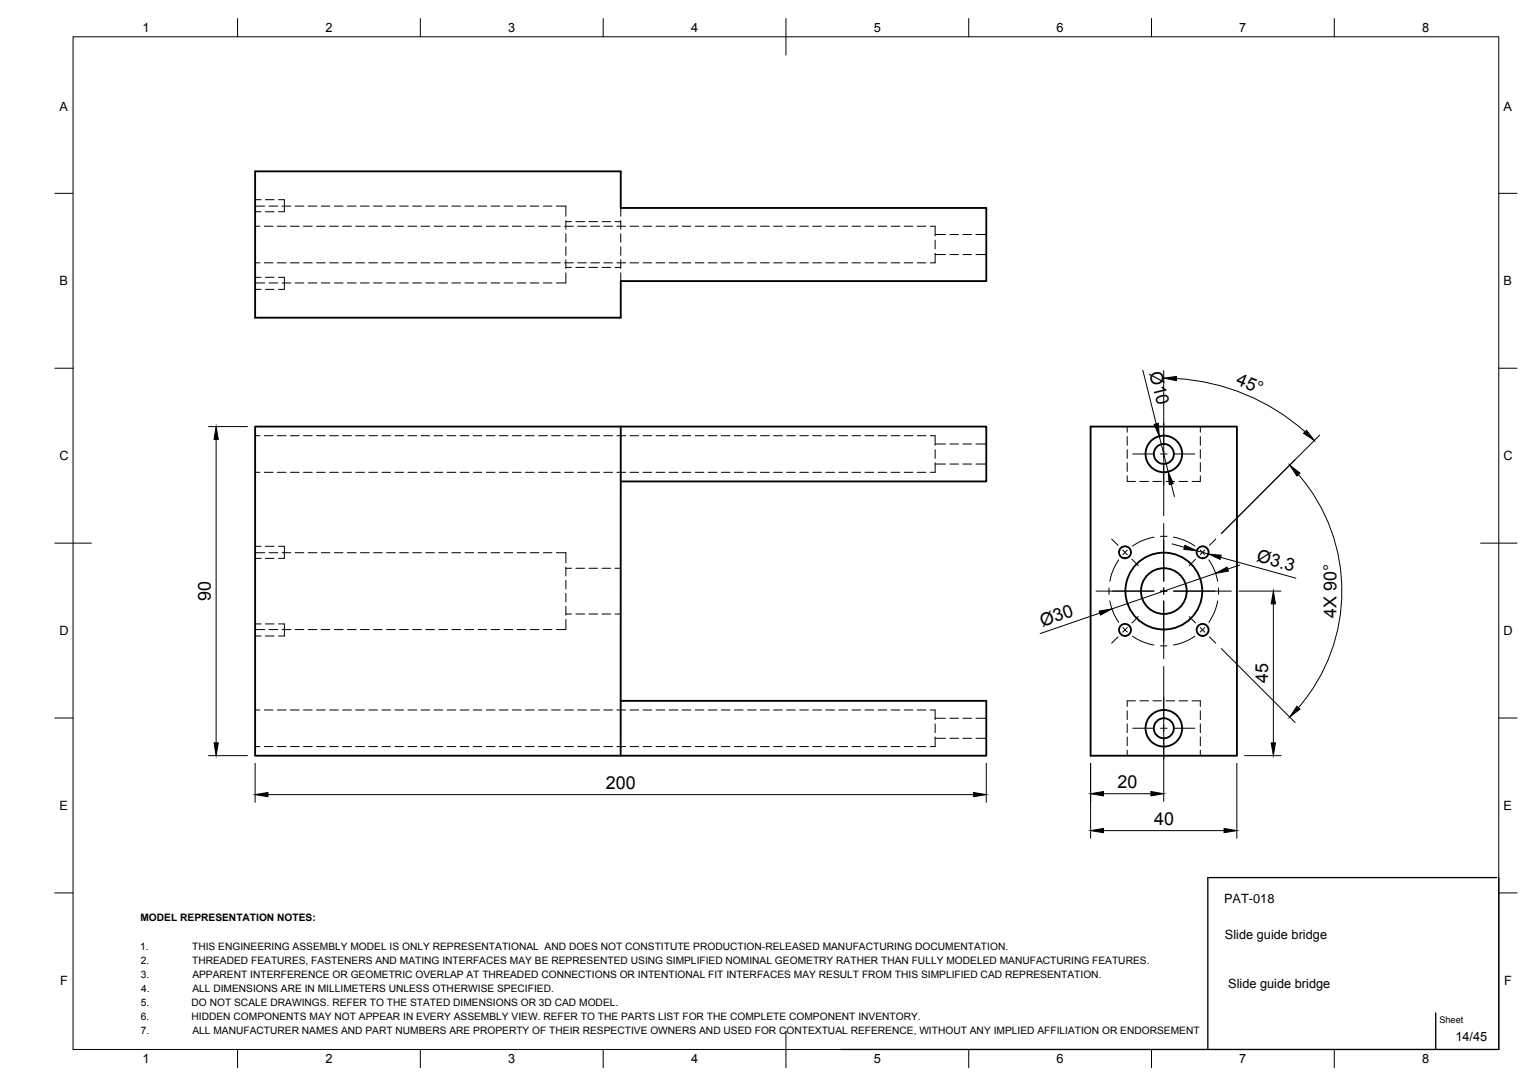
ISO-10303-21;
HEADER;
/* Generated by software containing ST-Developer
 * from STEP Tools, Inc. (www.steptools.com) 
 */

FILE_DESCRIPTION(
/* description */ ('Cam-driven reciprocating slide'),
/* implementation_level */ '2;1');

FILE_NAME(
/* name */ 'Slide guide bridge.step',
/* time_stamp */ '2026-10-28T03:25:20-07:00',
/* author */ (''),
/* organization */ (''),
/* preprocessor_version */ 'ST-DEVELOPER v20.2',
/* originating_system */ 'Autodesk Translation Framework v15.17.0.0',
/* authorisation */ '');

FILE_SCHEMA (('AUTOMOTIVE_DESIGN { 1 0 10303 214 3 1 1 }'));
ENDSEC;

DATA;
#10=MECHANICAL_DESIGN_GEOMETRIC_PRESENTATION_REPRESENTATION('',(#431),#13277);
#357=SHAPE_REPRESENTATION_RELATIONSHIP('SRR','None',#13450,#394);
#394=ADVANCED_BREP_SHAPE_REPRESENTATION('',(#475),#13245);
#431=STYLED_ITEM('',(#13713),#475);
#475=MANIFOLD_SOLID_BREP('Body1',#6407);
#592=FACE_BOUND('',#1478,.T.);
#593=FACE_BOUND('',#1482,.T.);
#594=FACE_BOUND('',#1486,.T.);
#595=FACE_BOUND('',#1489,.T.);
#596=FACE_BOUND('',#1495,.T.);
#597=FACE_BOUND('',#1503,.T.);
#598=FACE_BOUND('',#1504,.T.);
#599=FACE_BOUND('',#1505,.T.);
#600=FACE_BOUND('',#1506,.T.);
#601=FACE_BOUND('',#1507,.T.);
#602=FACE_BOUND('',#1508,.T.);
#603=FACE_BOUND('',#1509,.T.);
#604=FACE_BOUND('',#1511,.T.);
#736=PLANE('',#7067);
#737=PLANE('',#7071);
#738=PLANE('',#7075);
#739=PLANE('',#7079);
#740=PLANE('',#7083);
#741=PLANE('',#7090);
#742=PLANE('',#7097);
#743=PLANE('',#7101);
#744=PLANE('',#7102);
#745=PLANE('',#7103);
#746=PLANE('',#7104);
#747=PLANE('',#7105);
#748=PLANE('',#7106);
#749=PLANE('',#7107);
#750=PLANE('',#7108);
#751=PLANE('',#7109);
#752=PLANE('',#7110);
#753=PLANE('',#7111);
#754=PLANE('',#7112);
#755=PLANE('',#7113);
#756=PLANE('',#7114);
#1004=FACE_OUTER_BOUND('',#1468,.T.);
#1005=FACE_OUTER_BOUND('',#1469,.T.);
#1006=FACE_OUTER_BOUND('',#1470,.T.);
#1007=FACE_OUTER_BOUND('',#1471,.T.);
#1008=FACE_OUTER_BOUND('',#1472,.T.);
#1009=FACE_OUTER_BOUND('',#1473,.T.);
#1010=FACE_OUTER_BOUND('',#1474,.T.);
#1011=FACE_OUTER_BOUND('',#1475,.T.);
#1012=FACE_OUTER_BOUND('',#1476,.T.);
#1013=FACE_OUTER_BOUND('',#1477,.T.);
#1014=FACE_OUTER_BOUND('',#1479,.T.);
#1015=FACE_OUTER_BOUND('',#1480,.T.);
#1016=FACE_OUTER_BOUND('',#1481,.T.);
#1017=FACE_OUTER_BOUND('',#1483,.T.);
#1018=FACE_OUTER_BOUND('',#1484,.T.);
#1019=FACE_OUTER_BOUND('',#1485,.T.);
#1020=FACE_OUTER_BOUND('',#1487,.T.);
#1021=FACE_OUTER_BOUND('',#1488,.T.);
#1022=FACE_OUTER_BOUND('',#1490,.T.);
#1023=FACE_OUTER_BOUND('',#1491,.T.);
#1024=FACE_OUTER_BOUND('',#1492,.T.);
#1025=FACE_OUTER_BOUND('',#1493,.T.);
#1026=FACE_OUTER_BOUND('',#1494,.T.);
#1027=FACE_OUTER_BOUND('',#1496,.T.);
#1028=FACE_OUTER_BOUND('',#1497,.T.);
#1029=FACE_OUTER_BOUND('',#1498,.T.);
#1030=FACE_OUTER_BOUND('',#1499,.T.);
#1031=FACE_OUTER_BOUND('',#1500,.T.);
#1032=FACE_OUTER_BOUND('',#1501,.T.);
#1033=FACE_OUTER_BOUND('',#1502,.T.);
#1034=FACE_OUTER_BOUND('',#1510,.T.);
#1468=EDGE_LOOP('',(#4816,#4817,#4818,#4819));
#1469=EDGE_LOOP('',(#4820));
#1470=EDGE_LOOP('',(#4821,#4822,#4823,#4824));
#1471=EDGE_LOOP('',(#4825));
#1472=EDGE_LOOP('',(#4826,#4827,#4828,#4829));
#1473=EDGE_LOOP('',(#4830));
#1474=EDGE_LOOP('',(#4831,#4832,#4833,#4834));
#1475=EDGE_LOOP('',(#4835));
#1476=EDGE_LOOP('',(#4836,#4837,#4838,#4839));
#1477=EDGE_LOOP('',(#4840));
#1478=EDGE_LOOP('',(#4841));
#1479=EDGE_LOOP('',(#4842,#4843,#4844,#4845));
#1480=EDGE_LOOP('',(#4846,#4847,#4848,#4849));
#1481=EDGE_LOOP('',(#4850));
#1482=EDGE_LOOP('',(#4851));
#1483=EDGE_LOOP('',(#4852,#4853,#4854,#4855));
#1484=EDGE_LOOP('',(#4856,#4857,#4858,#4859));
#1485=EDGE_LOOP('',(#4860));
#1486=EDGE_LOOP('',(#4861));
#1487=EDGE_LOOP('',(#4862,#4863,#4864,#4865));
#1488=EDGE_LOOP('',(#4866,#4867,#4868,#4869,#4870,#4871,#4872,#4873,#4874,
#4875,#4876,#4877));
#1489=EDGE_LOOP('',(#4878));
#1490=EDGE_LOOP('',(#4879,#4880,#4881,#4882));
#1491=EDGE_LOOP('',(#4883,#4884,#4885,#4886));
#1492=EDGE_LOOP('',(#4887,#4888,#4889,#4890));
#1493=EDGE_LOOP('',(#4891,#4892,#4893,#4894));
#1494=EDGE_LOOP('',(#4895,#4896,#4897,#4898));
#1495=EDGE_LOOP('',(#4899));
#1496=EDGE_LOOP('',(#4900,#4901,#4902,#4903,#4904,#4905,#4906,#4907));
#1497=EDGE_LOOP('',(#4908,#4909,#4910,#4911));
#1498=EDGE_LOOP('',(#4912,#4913,#4914,#4915));
#1499=EDGE_LOOP('',(#4916,#4917,#4918,#4919));
#1500=EDGE_LOOP('',(#4920,#4921,#4922,#4923));
#1501=EDGE_LOOP('',(#4924,#4925,#4926,#4927,#4928,#4929,#4930,#4931));
#1502=EDGE_LOOP('',(#4932,#4933,#4934,#4935));
#1503=EDGE_LOOP('',(#4936));
#1504=EDGE_LOOP('',(#4937));
#1505=EDGE_LOOP('',(#4938));
#1506=EDGE_LOOP('',(#4939));
#1507=EDGE_LOOP('',(#4940));
#1508=EDGE_LOOP('',(#4941));
#1509=EDGE_LOOP('',(#4942));
#1510=EDGE_LOOP('',(#4943,#4944,#4945,#4946));
#1511=EDGE_LOOP('',(#4947));
#1977=LINE('',#10259,#2416);
#1978=LINE('',#10266,#2417);
#1979=LINE('',#10273,#2418);
#1980=LINE('',#10280,#2419);
#1981=LINE('',#10287,#2420);
#1982=LINE('',#10295,#2421);
#1983=LINE('',#10300,#2422);
#1984=LINE('',#10308,#2423);
#1985=LINE('',#10313,#2424);
#1986=LINE('',#10321,#2425);
#1987=LINE('',#10325,#2426);
#1988=LINE('',#10327,#2427);
#1989=LINE('',#10329,#2428);
#1990=LINE('',#10331,#2429);
#1991=LINE('',#10333,#2430);
#1992=LINE('',#10335,#2431);
#1993=LINE('',#10337,#2432);
#1994=LINE('',#10339,#2433);
#1995=LINE('',#10341,#2434);
#1996=LINE('',#10343,#2435);
#1997=LINE('',#10345,#2436);
#1998=LINE('',#10346,#2437);
#1999=LINE('',#10350,#2438);
#2000=LINE('',#10351,#2439);
#2001=LINE('',#10352,#2440);
#2002=LINE('',#10356,#2441);
#2003=LINE('',#10357,#2442);
#2004=LINE('',#10358,#2443);
#2005=LINE('',#10361,#2444);
#2006=LINE('',#10363,#2445);
#2007=LINE('',#10364,#2446);
#2008=LINE('',#10367,#2447);
#2009=LINE('',#10368,#2448);
#2010=LINE('',#10371,#2449);
#2011=LINE('',#10372,#2450);
#2012=LINE('',#10374,#2451);
#2013=LINE('',#10375,#2452);
#2014=LINE('',#10379,#2453);
#2015=LINE('',#10381,#2454);
#2016=LINE('',#10382,#2455);
#2017=LINE('',#10385,#2456);
#2018=LINE('',#10386,#2457);
#2019=LINE('',#10389,#2458);
#2020=LINE('',#10390,#2459);
#2021=LINE('',#10392,#2460);
#2022=LINE('',#10393,#2461);
#2416=VECTOR('',#8239,0.165);
#2417=VECTOR('',#8248,0.165);
#2418=VECTOR('',#8257,0.165);
#2419=VECTOR('',#8266,0.165);
#2420=VECTOR('',#8275,1.05);
#2421=VECTOR('',#8286,0.625);
#2422=VECTOR('',#8291,0.5);
#2423=VECTOR('',#8302,0.275);
#2424=VECTOR('',#8307,0.5);
#2425=VECTOR('',#8318,0.275);
#2426=VECTOR('',#8321,1.);
#2427=VECTOR('',#8322,1.);
#2428=VECTOR('',#8323,1.);
#2429=VECTOR('',#8324,1.);
#2430=VECTOR('',#8325,1.);
#2431=VECTOR('',#8326,1.);
#2432=VECTOR('',#8327,1.);
#2433=VECTOR('',#8328,1.);
#2434=VECTOR('',#8329,1.);
#2435=VECTOR('',#8330,1.);
#2436=VECTOR('',#8331,1.);
#2437=VECTOR('',#8332,1.);
#2438=VECTOR('',#8335,1.);
#2439=VECTOR('',#8336,1.);
#2440=VECTOR('',#8337,1.);
#2441=VECTOR('',#8340,1.);
#2442=VECTOR('',#8341,1.);
#2443=VECTOR('',#8342,1.);
#2444=VECTOR('',#8345,1.);
#2445=VECTOR('',#8346,1.);
#2446=VECTOR('',#8347,1.);
#2447=VECTOR('',#8350,1.);
#2448=VECTOR('',#8351,1.);
#2449=VECTOR('',#8354,1.);
#2450=VECTOR('',#8355,1.);
#2451=VECTOR('',#8358,1.);
#2452=VECTOR('',#8359,1.);
#2453=VECTOR('',#8364,1.);
#2454=VECTOR('',#8365,1.);
#2455=VECTOR('',#8366,1.);
#2456=VECTOR('',#8369,1.);
#2457=VECTOR('',#8370,1.);
#2458=VECTOR('',#8373,1.);
#2459=VECTOR('',#8374,1.);
#2460=VECTOR('',#8377,1.);
#2461=VECTOR('',#8378,1.);
#2807=CIRCLE('',#7065,0.165);
#2808=CIRCLE('',#7066,0.165);
#2809=CIRCLE('',#7069,0.165);
#2810=CIRCLE('',#7070,0.165);
#2811=CIRCLE('',#7073,0.165);
#2812=CIRCLE('',#7074,0.165);
#2813=CIRCLE('',#7077,0.165);
#2814=CIRCLE('',#7078,0.165);
#2815=CIRCLE('',#7081,1.05);
#2816=CIRCLE('',#7082,1.05);
#2817=CIRCLE('',#7084,0.625);
#2818=CIRCLE('',#7086,0.625);
#2819=CIRCLE('',#7088,0.5);
#2820=CIRCLE('',#7089,0.5);
#2821=CIRCLE('',#7091,0.275);
#2822=CIRCLE('',#7093,0.275);
#2823=CIRCLE('',#7095,0.5);
#2824=CIRCLE('',#7096,0.5);
#2825=CIRCLE('',#7098,0.275);
#2826=CIRCLE('',#7100,0.275);
#3195=VERTEX_POINT('',#10256);
#3196=VERTEX_POINT('',#10258);
#3197=VERTEX_POINT('',#10263);
#3198=VERTEX_POINT('',#10265);
#3199=VERTEX_POINT('',#10270);
#3200=VERTEX_POINT('',#10272);
#3201=VERTEX_POINT('',#10277);
#3202=VERTEX_POINT('',#10279);
#3203=VERTEX_POINT('',#10284);
#3204=VERTEX_POINT('',#10286);
#3205=VERTEX_POINT('',#10290);
#3206=VERTEX_POINT('',#10293);
#3207=VERTEX_POINT('',#10297);
#3208=VERTEX_POINT('',#10299);
#3209=VERTEX_POINT('',#10303);
#3210=VERTEX_POINT('',#10306);
#3211=VERTEX_POINT('',#10310);
#3212=VERTEX_POINT('',#10312);
#3213=VERTEX_POINT('',#10316);
#3214=VERTEX_POINT('',#10319);
#3215=VERTEX_POINT('',#10323);
#3216=VERTEX_POINT('',#10324);
#3217=VERTEX_POINT('',#10326);
#3218=VERTEX_POINT('',#10328);
#3219=VERTEX_POINT('',#10330);
#3220=VERTEX_POINT('',#10332);
#3221=VERTEX_POINT('',#10334);
#3222=VERTEX_POINT('',#10336);
#3223=VERTEX_POINT('',#10338);
#3224=VERTEX_POINT('',#10340);
#3225=VERTEX_POINT('',#10342);
#3226=VERTEX_POINT('',#10344);
#3227=VERTEX_POINT('',#10348);
#3228=VERTEX_POINT('',#10349);
#3229=VERTEX_POINT('',#10354);
#3230=VERTEX_POINT('',#10355);
#3231=VERTEX_POINT('',#10360);
#3232=VERTEX_POINT('',#10362);
#3233=VERTEX_POINT('',#10366);
#3234=VERTEX_POINT('',#10370);
#3235=VERTEX_POINT('',#10378);
#3236=VERTEX_POINT('',#10380);
#3237=VERTEX_POINT('',#10384);
#3238=VERTEX_POINT('',#10388);
#3798=EDGE_CURVE('',#3195,#3195,#2807,.T.);
#3799=EDGE_CURVE('',#3195,#3196,#1977,.T.);
#3800=EDGE_CURVE('',#3196,#3196,#2808,.T.);
#3801=EDGE_CURVE('',#3197,#3197,#2809,.T.);
#3802=EDGE_CURVE('',#3197,#3198,#1978,.T.);
#3803=EDGE_CURVE('',#3198,#3198,#2810,.T.);
#3804=EDGE_CURVE('',#3199,#3199,#2811,.T.);
#3805=EDGE_CURVE('',#3199,#3200,#1979,.T.);
#3806=EDGE_CURVE('',#3200,#3200,#2812,.T.);
#3807=EDGE_CURVE('',#3201,#3201,#2813,.T.);
#3808=EDGE_CURVE('',#3201,#3202,#1980,.T.);
#3809=EDGE_CURVE('',#3202,#3202,#2814,.T.);
#3810=EDGE_CURVE('',#3203,#3203,#2815,.T.);
#3811=EDGE_CURVE('',#3203,#3204,#1981,.T.);
#3812=EDGE_CURVE('',#3204,#3204,#2816,.T.);
#3813=EDGE_CURVE('',#3205,#3205,#2817,.T.);
#3814=EDGE_CURVE('',#3206,#3206,#2818,.T.);
#3815=EDGE_CURVE('',#3206,#3205,#1982,.T.);
#3816=EDGE_CURVE('',#3207,#3207,#2819,.T.);
#3817=EDGE_CURVE('',#3207,#3208,#1983,.T.);
#3818=EDGE_CURVE('',#3208,#3208,#2820,.T.);
#3819=EDGE_CURVE('',#3209,#3209,#2821,.T.);
#3820=EDGE_CURVE('',#3210,#3210,#2822,.T.);
#3821=EDGE_CURVE('',#3210,#3209,#1984,.T.);
#3822=EDGE_CURVE('',#3211,#3211,#2823,.T.);
#3823=EDGE_CURVE('',#3211,#3212,#1985,.T.);
#3824=EDGE_CURVE('',#3212,#3212,#2824,.T.);
#3825=EDGE_CURVE('',#3213,#3213,#2825,.T.);
#3826=EDGE_CURVE('',#3214,#3214,#2826,.T.);
#3827=EDGE_CURVE('',#3214,#3213,#1986,.T.);
#3828=EDGE_CURVE('',#3215,#3216,#1987,.T.);
#3829=EDGE_CURVE('',#3215,#3217,#1988,.T.);
#3830=EDGE_CURVE('',#3218,#3217,#1989,.T.);
#3831=EDGE_CURVE('',#3219,#3218,#1990,.T.);
#3832=EDGE_CURVE('',#3220,#3219,#1991,.T.);
#3833=EDGE_CURVE('',#3221,#3220,#1992,.T.);
#3834=EDGE_CURVE('',#3222,#3221,#1993,.T.);
#3835=EDGE_CURVE('',#3223,#3222,#1994,.T.);
#3836=EDGE_CURVE('',#3224,#3223,#1995,.T.);
#3837=EDGE_CURVE('',#3224,#3225,#1996,.T.);
#3838=EDGE_CURVE('',#3226,#3225,#1997,.T.);
#3839=EDGE_CURVE('',#3216,#3226,#1998,.T.);
#3840=EDGE_CURVE('',#3227,#3228,#1999,.T.);
#3841=EDGE_CURVE('',#3228,#3218,#2000,.T.);
#3842=EDGE_CURVE('',#3217,#3227,#2001,.T.);
#3843=EDGE_CURVE('',#3229,#3230,#2002,.T.);
#3844=EDGE_CURVE('',#3230,#3224,#2003,.T.);
#3845=EDGE_CURVE('',#3223,#3229,#2004,.T.);
#3846=EDGE_CURVE('',#3231,#3220,#2005,.T.);
#3847=EDGE_CURVE('',#3232,#3231,#2006,.T.);
#3848=EDGE_CURVE('',#3221,#3232,#2007,.T.);
#3849=EDGE_CURVE('',#3219,#3233,#2008,.T.);
#3850=EDGE_CURVE('',#3233,#3231,#2009,.T.);
#3851=EDGE_CURVE('',#3232,#3234,#2010,.T.);
#3852=EDGE_CURVE('',#3234,#3233,#2011,.T.);
#3853=EDGE_CURVE('',#3234,#3222,#2012,.T.);
#3854=EDGE_CURVE('',#3229,#3228,#2013,.T.);
#3855=EDGE_CURVE('',#3235,#3226,#2014,.T.);
#3856=EDGE_CURVE('',#3235,#3236,#2015,.T.);
#3857=EDGE_CURVE('',#3236,#3216,#2016,.T.);
#3858=EDGE_CURVE('',#3237,#3225,#2017,.T.);
#3859=EDGE_CURVE('',#3237,#3235,#2018,.T.);
#3860=EDGE_CURVE('',#3236,#3238,#2019,.T.);
#3861=EDGE_CURVE('',#3238,#3215,#2020,.T.);
#3862=EDGE_CURVE('',#3238,#3237,#2021,.T.);
#3863=EDGE_CURVE('',#3230,#3227,#2022,.T.);
#4816=ORIENTED_EDGE('',*,*,#3798,.F.);
#4817=ORIENTED_EDGE('',*,*,#3799,.T.);
#4818=ORIENTED_EDGE('',*,*,#3800,.F.);
#4819=ORIENTED_EDGE('',*,*,#3799,.F.);
#4820=ORIENTED_EDGE('',*,*,#3798,.T.);
#4821=ORIENTED_EDGE('',*,*,#3801,.F.);
#4822=ORIENTED_EDGE('',*,*,#3802,.T.);
#4823=ORIENTED_EDGE('',*,*,#3803,.F.);
#4824=ORIENTED_EDGE('',*,*,#3802,.F.);
#4825=ORIENTED_EDGE('',*,*,#3801,.T.);
#4826=ORIENTED_EDGE('',*,*,#3804,.F.);
#4827=ORIENTED_EDGE('',*,*,#3805,.T.);
#4828=ORIENTED_EDGE('',*,*,#3806,.F.);
#4829=ORIENTED_EDGE('',*,*,#3805,.F.);
#4830=ORIENTED_EDGE('',*,*,#3804,.T.);
#4831=ORIENTED_EDGE('',*,*,#3807,.F.);
#4832=ORIENTED_EDGE('',*,*,#3808,.T.);
#4833=ORIENTED_EDGE('',*,*,#3809,.F.);
#4834=ORIENTED_EDGE('',*,*,#3808,.F.);
#4835=ORIENTED_EDGE('',*,*,#3807,.T.);
#4836=ORIENTED_EDGE('',*,*,#3810,.F.);
#4837=ORIENTED_EDGE('',*,*,#3811,.T.);
#4838=ORIENTED_EDGE('',*,*,#3812,.F.);
#4839=ORIENTED_EDGE('',*,*,#3811,.F.);
#4840=ORIENTED_EDGE('',*,*,#3810,.T.);
#4841=ORIENTED_EDGE('',*,*,#3813,.F.);
#4842=ORIENTED_EDGE('',*,*,#3814,.F.);
#4843=ORIENTED_EDGE('',*,*,#3815,.T.);
#4844=ORIENTED_EDGE('',*,*,#3813,.T.);
#4845=ORIENTED_EDGE('',*,*,#3815,.F.);
#4846=ORIENTED_EDGE('',*,*,#3816,.F.);
#4847=ORIENTED_EDGE('',*,*,#3817,.T.);
#4848=ORIENTED_EDGE('',*,*,#3818,.F.);
#4849=ORIENTED_EDGE('',*,*,#3817,.F.);
#4850=ORIENTED_EDGE('',*,*,#3816,.T.);
#4851=ORIENTED_EDGE('',*,*,#3819,.F.);
#4852=ORIENTED_EDGE('',*,*,#3820,.F.);
#4853=ORIENTED_EDGE('',*,*,#3821,.T.);
#4854=ORIENTED_EDGE('',*,*,#3819,.T.);
#4855=ORIENTED_EDGE('',*,*,#3821,.F.);
#4856=ORIENTED_EDGE('',*,*,#3822,.F.);
#4857=ORIENTED_EDGE('',*,*,#3823,.T.);
#4858=ORIENTED_EDGE('',*,*,#3824,.F.);
#4859=ORIENTED_EDGE('',*,*,#3823,.F.);
#4860=ORIENTED_EDGE('',*,*,#3822,.T.);
#4861=ORIENTED_EDGE('',*,*,#3825,.F.);
#4862=ORIENTED_EDGE('',*,*,#3826,.F.);
#4863=ORIENTED_EDGE('',*,*,#3827,.T.);
#4864=ORIENTED_EDGE('',*,*,#3825,.T.);
#4865=ORIENTED_EDGE('',*,*,#3827,.F.);
#4866=ORIENTED_EDGE('',*,*,#3828,.F.);
#4867=ORIENTED_EDGE('',*,*,#3829,.T.);
#4868=ORIENTED_EDGE('',*,*,#3830,.F.);
#4869=ORIENTED_EDGE('',*,*,#3831,.F.);
#4870=ORIENTED_EDGE('',*,*,#3832,.F.);
#4871=ORIENTED_EDGE('',*,*,#3833,.F.);
#4872=ORIENTED_EDGE('',*,*,#3834,.F.);
#4873=ORIENTED_EDGE('',*,*,#3835,.F.);
#4874=ORIENTED_EDGE('',*,*,#3836,.F.);
#4875=ORIENTED_EDGE('',*,*,#3837,.T.);
#4876=ORIENTED_EDGE('',*,*,#3838,.F.);
#4877=ORIENTED_EDGE('',*,*,#3839,.F.);
#4878=ORIENTED_EDGE('',*,*,#3814,.T.);
#4879=ORIENTED_EDGE('',*,*,#3840,.T.);
#4880=ORIENTED_EDGE('',*,*,#3841,.T.);
#4881=ORIENTED_EDGE('',*,*,#3830,.T.);
#4882=ORIENTED_EDGE('',*,*,#3842,.T.);
#4883=ORIENTED_EDGE('',*,*,#3843,.T.);
#4884=ORIENTED_EDGE('',*,*,#3844,.T.);
#4885=ORIENTED_EDGE('',*,*,#3836,.T.);
#4886=ORIENTED_EDGE('',*,*,#3845,.T.);
#4887=ORIENTED_EDGE('',*,*,#3833,.T.);
#4888=ORIENTED_EDGE('',*,*,#3846,.F.);
#4889=ORIENTED_EDGE('',*,*,#3847,.F.);
#4890=ORIENTED_EDGE('',*,*,#3848,.F.);
#4891=ORIENTED_EDGE('',*,*,#3832,.T.);
#4892=ORIENTED_EDGE('',*,*,#3849,.T.);
#4893=ORIENTED_EDGE('',*,*,#3850,.T.);
#4894=ORIENTED_EDGE('',*,*,#3846,.T.);
#4895=ORIENTED_EDGE('',*,*,#3851,.F.);
#4896=ORIENTED_EDGE('',*,*,#3847,.T.);
#4897=ORIENTED_EDGE('',*,*,#3850,.F.);
#4898=ORIENTED_EDGE('',*,*,#3852,.F.);
#4899=ORIENTED_EDGE('',*,*,#3820,.T.);
#4900=ORIENTED_EDGE('',*,*,#3853,.F.);
#4901=ORIENTED_EDGE('',*,*,#3852,.T.);
#4902=ORIENTED_EDGE('',*,*,#3849,.F.);
#4903=ORIENTED_EDGE('',*,*,#3831,.T.);
#4904=ORIENTED_EDGE('',*,*,#3841,.F.);
#4905=ORIENTED_EDGE('',*,*,#3854,.F.);
#4906=ORIENTED_EDGE('',*,*,#3845,.F.);
#4907=ORIENTED_EDGE('',*,*,#3835,.T.);
#4908=ORIENTED_EDGE('',*,*,#3834,.T.);
#4909=ORIENTED_EDGE('',*,*,#3848,.T.);
#4910=ORIENTED_EDGE('',*,*,#3851,.T.);
#4911=ORIENTED_EDGE('',*,*,#3853,.T.);
#4912=ORIENTED_EDGE('',*,*,#3839,.T.);
#4913=ORIENTED_EDGE('',*,*,#3855,.F.);
#4914=ORIENTED_EDGE('',*,*,#3856,.T.);
#4915=ORIENTED_EDGE('',*,*,#3857,.T.);
#4916=ORIENTED_EDGE('',*,*,#3838,.T.);
#4917=ORIENTED_EDGE('',*,*,#3858,.F.);
#4918=ORIENTED_EDGE('',*,*,#3859,.T.);
#4919=ORIENTED_EDGE('',*,*,#3855,.T.);
#4920=ORIENTED_EDGE('',*,*,#3828,.T.);
#4921=ORIENTED_EDGE('',*,*,#3857,.F.);
#4922=ORIENTED_EDGE('',*,*,#3860,.T.);
#4923=ORIENTED_EDGE('',*,*,#3861,.T.);
#4924=ORIENTED_EDGE('',*,*,#3861,.F.);
#4925=ORIENTED_EDGE('',*,*,#3862,.T.);
#4926=ORIENTED_EDGE('',*,*,#3858,.T.);
#4927=ORIENTED_EDGE('',*,*,#3837,.F.);
#4928=ORIENTED_EDGE('',*,*,#3844,.F.);
#4929=ORIENTED_EDGE('',*,*,#3863,.T.);
#4930=ORIENTED_EDGE('',*,*,#3842,.F.);
#4931=ORIENTED_EDGE('',*,*,#3829,.F.);
#4932=ORIENTED_EDGE('',*,*,#3863,.F.);
#4933=ORIENTED_EDGE('',*,*,#3843,.F.);
#4934=ORIENTED_EDGE('',*,*,#3854,.T.);
#4935=ORIENTED_EDGE('',*,*,#3840,.F.);
#4936=ORIENTED_EDGE('',*,*,#3824,.T.);
#4937=ORIENTED_EDGE('',*,*,#3818,.T.);
#4938=ORIENTED_EDGE('',*,*,#3812,.T.);
#4939=ORIENTED_EDGE('',*,*,#3809,.T.);
#4940=ORIENTED_EDGE('',*,*,#3806,.T.);
#4941=ORIENTED_EDGE('',*,*,#3803,.T.);
#4942=ORIENTED_EDGE('',*,*,#3800,.T.);
#4943=ORIENTED_EDGE('',*,*,#3862,.F.);
#4944=ORIENTED_EDGE('',*,*,#3860,.F.);
#4945=ORIENTED_EDGE('',*,*,#3856,.F.);
#4946=ORIENTED_EDGE('',*,*,#3859,.F.);
#4947=ORIENTED_EDGE('',*,*,#3826,.T.);
#5940=CYLINDRICAL_SURFACE('',#7064,0.165);
#5941=CYLINDRICAL_SURFACE('',#7068,0.165);
#5942=CYLINDRICAL_SURFACE('',#7072,0.165);
#5943=CYLINDRICAL_SURFACE('',#7076,0.165);
#5944=CYLINDRICAL_SURFACE('',#7080,1.05);
#5945=CYLINDRICAL_SURFACE('',#7085,0.625);
#5946=CYLINDRICAL_SURFACE('',#7087,0.5);
#5947=CYLINDRICAL_SURFACE('',#7092,0.275);
#5948=CYLINDRICAL_SURFACE('',#7094,0.5);
#5949=CYLINDRICAL_SURFACE('',#7099,0.275);
#6122=ADVANCED_FACE('',(#1004),#5940,.F.);
#6123=ADVANCED_FACE('',(#1005),#736,.T.);
#6124=ADVANCED_FACE('',(#1006),#5941,.F.);
#6125=ADVANCED_FACE('',(#1007),#737,.T.);
#6126=ADVANCED_FACE('',(#1008),#5942,.F.);
#6127=ADVANCED_FACE('',(#1009),#738,.T.);
#6128=ADVANCED_FACE('',(#1010),#5943,.F.);
#6129=ADVANCED_FACE('',(#1011),#739,.T.);
#6130=ADVANCED_FACE('',(#1012),#5944,.F.);
#6131=ADVANCED_FACE('',(#1013,#592),#740,.T.);
#6132=ADVANCED_FACE('',(#1014),#5945,.F.);
#6133=ADVANCED_FACE('',(#1015),#5946,.F.);
#6134=ADVANCED_FACE('',(#1016,#593),#741,.T.);
#6135=ADVANCED_FACE('',(#1017),#5947,.F.);
#6136=ADVANCED_FACE('',(#1018),#5948,.F.);
#6137=ADVANCED_FACE('',(#1019,#594),#742,.T.);
#6138=ADVANCED_FACE('',(#1020),#5949,.F.);
#6139=ADVANCED_FACE('',(#1021,#595),#743,.T.);
#6140=ADVANCED_FACE('',(#1022),#744,.T.);
#6141=ADVANCED_FACE('',(#1023),#745,.F.);
#6142=ADVANCED_FACE('',(#1024),#746,.T.);
#6143=ADVANCED_FACE('',(#1025),#747,.T.);
#6144=ADVANCED_FACE('',(#1026,#596),#748,.T.);
#6145=ADVANCED_FACE('',(#1027),#749,.T.);
#6146=ADVANCED_FACE('',(#1028),#750,.F.);
#6147=ADVANCED_FACE('',(#1029),#751,.T.);
#6148=ADVANCED_FACE('',(#1030),#752,.T.);
#6149=ADVANCED_FACE('',(#1031),#753,.T.);
#6150=ADVANCED_FACE('',(#1032),#754,.T.);
#6151=ADVANCED_FACE('',(#1033,#597,#598,#599,#600,#601,#602,#603),#755,
 .T.);
#6152=ADVANCED_FACE('',(#1034,#604),#756,.F.);
#6407=CLOSED_SHELL('',(#6122,#6123,#6124,#6125,#6126,#6127,#6128,#6129,
#6130,#6131,#6132,#6133,#6134,#6135,#6136,#6137,#6138,#6139,#6140,#6141,
#6142,#6143,#6144,#6145,#6146,#6147,#6148,#6149,#6150,#6151,#6152));
#7063=AXIS2_PLACEMENT_3D('',#10254,#8233,#8234);
#7064=AXIS2_PLACEMENT_3D('',#10255,#8235,#8236);
#7065=AXIS2_PLACEMENT_3D('',#10257,#8237,#8238);
#7066=AXIS2_PLACEMENT_3D('',#10260,#8240,#8241);
#7067=AXIS2_PLACEMENT_3D('',#10261,#8242,#8243);
#7068=AXIS2_PLACEMENT_3D('',#10262,#8244,#8245);
#7069=AXIS2_PLACEMENT_3D('',#10264,#8246,#8247);
#7070=AXIS2_PLACEMENT_3D('',#10267,#8249,#8250);
#7071=AXIS2_PLACEMENT_3D('',#10268,#8251,#8252);
#7072=AXIS2_PLACEMENT_3D('',#10269,#8253,#8254);
#7073=AXIS2_PLACEMENT_3D('',#10271,#8255,#8256);
#7074=AXIS2_PLACEMENT_3D('',#10274,#8258,#8259);
#7075=AXIS2_PLACEMENT_3D('',#10275,#8260,#8261);
#7076=AXIS2_PLACEMENT_3D('',#10276,#8262,#8263);
#7077=AXIS2_PLACEMENT_3D('',#10278,#8264,#8265);
#7078=AXIS2_PLACEMENT_3D('',#10281,#8267,#8268);
#7079=AXIS2_PLACEMENT_3D('',#10282,#8269,#8270);
#7080=AXIS2_PLACEMENT_3D('',#10283,#8271,#8272);
#7081=AXIS2_PLACEMENT_3D('',#10285,#8273,#8274);
#7082=AXIS2_PLACEMENT_3D('',#10288,#8276,#8277);
#7083=AXIS2_PLACEMENT_3D('',#10289,#8278,#8279);
#7084=AXIS2_PLACEMENT_3D('',#10291,#8280,#8281);
#7085=AXIS2_PLACEMENT_3D('',#10292,#8282,#8283);
#7086=AXIS2_PLACEMENT_3D('',#10294,#8284,#8285);
#7087=AXIS2_PLACEMENT_3D('',#10296,#8287,#8288);
#7088=AXIS2_PLACEMENT_3D('',#10298,#8289,#8290);
#7089=AXIS2_PLACEMENT_3D('',#10301,#8292,#8293);
#7090=AXIS2_PLACEMENT_3D('',#10302,#8294,#8295);
#7091=AXIS2_PLACEMENT_3D('',#10304,#8296,#8297);
#7092=AXIS2_PLACEMENT_3D('',#10305,#8298,#8299);
#7093=AXIS2_PLACEMENT_3D('',#10307,#8300,#8301);
#7094=AXIS2_PLACEMENT_3D('',#10309,#8303,#8304);
#7095=AXIS2_PLACEMENT_3D('',#10311,#8305,#8306);
#7096=AXIS2_PLACEMENT_3D('',#10314,#8308,#8309);
#7097=AXIS2_PLACEMENT_3D('',#10315,#8310,#8311);
#7098=AXIS2_PLACEMENT_3D('',#10317,#8312,#8313);
#7099=AXIS2_PLACEMENT_3D('',#10318,#8314,#8315);
#7100=AXIS2_PLACEMENT_3D('',#10320,#8316,#8317);
#7101=AXIS2_PLACEMENT_3D('',#10322,#8319,#8320);
#7102=AXIS2_PLACEMENT_3D('',#10347,#8333,#8334);
#7103=AXIS2_PLACEMENT_3D('',#10353,#8338,#8339);
#7104=AXIS2_PLACEMENT_3D('',#10359,#8343,#8344);
#7105=AXIS2_PLACEMENT_3D('',#10365,#8348,#8349);
#7106=AXIS2_PLACEMENT_3D('',#10369,#8352,#8353);
#7107=AXIS2_PLACEMENT_3D('',#10373,#8356,#8357);
#7108=AXIS2_PLACEMENT_3D('',#10376,#8360,#8361);
#7109=AXIS2_PLACEMENT_3D('',#10377,#8362,#8363);
#7110=AXIS2_PLACEMENT_3D('',#10383,#8367,#8368);
#7111=AXIS2_PLACEMENT_3D('',#10387,#8371,#8372);
#7112=AXIS2_PLACEMENT_3D('',#10391,#8375,#8376);
#7113=AXIS2_PLACEMENT_3D('',#10394,#8379,#8380);
#7114=AXIS2_PLACEMENT_3D('',#10395,#8381,#8382);
#8233=DIRECTION('axis',(0.,0.,1.));
#8234=DIRECTION('refdir',(1.,0.,0.));
#8235=DIRECTION('center_axis',(0.,0.,1.));
#8236=DIRECTION('ref_axis',(1.,0.,0.));
#8237=DIRECTION('center_axis',(0.,0.,1.));
#8238=DIRECTION('ref_axis',(1.,0.,0.));
#8239=DIRECTION('',(0.,0.,1.));
#8240=DIRECTION('center_axis',(0.,0.,-1.));
#8241=DIRECTION('ref_axis',(1.,0.,0.));
#8242=DIRECTION('center_axis',(0.,0.,1.));
#8243=DIRECTION('ref_axis',(1.,0.,0.));
#8244=DIRECTION('center_axis',(0.,0.,1.));
#8245=DIRECTION('ref_axis',(1.,0.,0.));
#8246=DIRECTION('center_axis',(0.,0.,1.));
#8247=DIRECTION('ref_axis',(1.,0.,0.));
#8248=DIRECTION('',(0.,0.,1.));
#8249=DIRECTION('center_axis',(0.,0.,-1.));
#8250=DIRECTION('ref_axis',(1.,0.,0.));
#8251=DIRECTION('center_axis',(0.,0.,1.));
#8252=DIRECTION('ref_axis',(1.,0.,0.));
#8253=DIRECTION('center_axis',(0.,0.,1.));
#8254=DIRECTION('ref_axis',(1.,0.,0.));
#8255=DIRECTION('center_axis',(0.,0.,1.));
#8256=DIRECTION('ref_axis',(1.,0.,0.));
#8257=DIRECTION('',(0.,0.,1.));
#8258=DIRECTION('center_axis',(0.,0.,-1.));
#8259=DIRECTION('ref_axis',(1.,0.,0.));
#8260=DIRECTION('center_axis',(0.,0.,1.));
#8261=DIRECTION('ref_axis',(1.,0.,0.));
#8262=DIRECTION('center_axis',(0.,0.,1.));
#8263=DIRECTION('ref_axis',(1.,0.,0.));
#8264=DIRECTION('center_axis',(0.,0.,1.));
#8265=DIRECTION('ref_axis',(1.,0.,0.));
#8266=DIRECTION('',(0.,0.,1.));
#8267=DIRECTION('center_axis',(0.,0.,-1.));
#8268=DIRECTION('ref_axis',(1.,0.,0.));
#8269=DIRECTION('center_axis',(0.,0.,1.));
#8270=DIRECTION('ref_axis',(1.,0.,0.));
#8271=DIRECTION('center_axis',(0.,0.,1.));
#8272=DIRECTION('ref_axis',(1.,0.,0.));
#8273=DIRECTION('center_axis',(0.,0.,1.));
#8274=DIRECTION('ref_axis',(1.,0.,0.));
#8275=DIRECTION('',(0.,0.,1.));
#8276=DIRECTION('center_axis',(0.,0.,-1.));
#8277=DIRECTION('ref_axis',(1.,0.,0.));
#8278=DIRECTION('center_axis',(0.,0.,1.));
#8279=DIRECTION('ref_axis',(1.,0.,0.));
#8280=DIRECTION('center_axis',(0.,0.,1.));
#8281=DIRECTION('ref_axis',(1.,0.,0.));
#8282=DIRECTION('center_axis',(0.,0.,1.));
#8283=DIRECTION('ref_axis',(1.,0.,0.));
#8284=DIRECTION('center_axis',(0.,0.,1.));
#8285=DIRECTION('ref_axis',(1.,0.,0.));
#8286=DIRECTION('',(0.,0.,1.));
#8287=DIRECTION('center_axis',(0.,0.,1.));
#8288=DIRECTION('ref_axis',(1.,0.,0.));
#8289=DIRECTION('center_axis',(0.,0.,1.));
#8290=DIRECTION('ref_axis',(1.,0.,0.));
#8291=DIRECTION('',(0.,0.,1.));
#8292=DIRECTION('center_axis',(0.,0.,-1.));
#8293=DIRECTION('ref_axis',(1.,0.,0.));
#8294=DIRECTION('center_axis',(0.,0.,1.));
#8295=DIRECTION('ref_axis',(1.,0.,0.));
#8296=DIRECTION('center_axis',(0.,0.,1.));
#8297=DIRECTION('ref_axis',(1.,0.,0.));
#8298=DIRECTION('center_axis',(0.,0.,1.));
#8299=DIRECTION('ref_axis',(1.,0.,0.));
#8300=DIRECTION('center_axis',(0.,0.,1.));
#8301=DIRECTION('ref_axis',(1.,0.,0.));
#8302=DIRECTION('',(0.,0.,1.));
#8303=DIRECTION('center_axis',(0.,0.,1.));
#8304=DIRECTION('ref_axis',(1.,0.,0.));
#8305=DIRECTION('center_axis',(0.,0.,1.));
#8306=DIRECTION('ref_axis',(1.,0.,0.));
#8307=DIRECTION('',(0.,0.,1.));
#8308=DIRECTION('center_axis',(0.,0.,-1.));
#8309=DIRECTION('ref_axis',(1.,0.,0.));
#8310=DIRECTION('center_axis',(0.,0.,1.));
#8311=DIRECTION('ref_axis',(1.,0.,0.));
#8312=DIRECTION('center_axis',(0.,0.,1.));
#8313=DIRECTION('ref_axis',(1.,0.,0.));
#8314=DIRECTION('center_axis',(0.,0.,1.));
#8315=DIRECTION('ref_axis',(1.,0.,0.));
#8316=DIRECTION('center_axis',(0.,0.,1.));
#8317=DIRECTION('ref_axis',(1.,0.,0.));
#8318=DIRECTION('',(0.,0.,1.));
#8319=DIRECTION('center_axis',(0.,0.,-1.));
#8320=DIRECTION('ref_axis',(-1.,0.,0.));
#8321=DIRECTION('',(1.,0.,0.));
#8322=DIRECTION('',(0.,1.,0.));
#8323=DIRECTION('',(-1.,0.,0.));
#8324=DIRECTION('',(0.,1.,0.));
#8325=DIRECTION('',(1.,0.,0.));
#8326=DIRECTION('',(0.,1.,0.));
#8327=DIRECTION('',(-1.,0.,0.));
#8328=DIRECTION('',(0.,1.,0.));
#8329=DIRECTION('',(1.,0.,0.));
#8330=DIRECTION('',(0.,1.,0.));
#8331=DIRECTION('',(-1.,0.,0.));
#8332=DIRECTION('',(0.,-1.,0.));
#8333=DIRECTION('center_axis',(0.,1.,0.));
#8334=DIRECTION('ref_axis',(0.,0.,1.));
#8335=DIRECTION('',(1.,0.,0.));
#8336=DIRECTION('',(0.,0.,-1.));
#8337=DIRECTION('',(0.,0.,1.));
#8338=DIRECTION('center_axis',(0.,1.,0.));
#8339=DIRECTION('ref_axis',(1.,0.,0.));
#8340=DIRECTION('',(-1.,0.,0.));
#8341=DIRECTION('',(0.,0.,-1.));
#8342=DIRECTION('',(0.,0.,1.));
#8343=DIRECTION('center_axis',(-1.,0.,0.));
#8344=DIRECTION('ref_axis',(0.,0.,1.));
#8345=DIRECTION('',(0.,0.,1.));
#8346=DIRECTION('',(0.,1.,0.));
#8347=DIRECTION('',(0.,0.,-1.));
#8348=DIRECTION('center_axis',(0.,1.,0.));
#8349=DIRECTION('ref_axis',(0.,0.,1.));
#8350=DIRECTION('',(0.,0.,-1.));
#8351=DIRECTION('',(-1.,0.,0.));
#8352=DIRECTION('center_axis',(0.,0.,-1.));
#8353=DIRECTION('ref_axis',(-1.,0.,0.));
#8354=DIRECTION('',(1.,0.,0.));
#8355=DIRECTION('',(0.,1.,0.));
#8356=DIRECTION('center_axis',(1.,0.,0.));
#8357=DIRECTION('ref_axis',(0.,0.,-1.));
#8358=DIRECTION('',(0.,0.,1.));
#8359=DIRECTION('',(0.,1.,0.));
#8360=DIRECTION('center_axis',(0.,1.,0.));
#8361=DIRECTION('ref_axis',(1.,0.,0.));
#8362=DIRECTION('center_axis',(1.,0.,0.));
#8363=DIRECTION('ref_axis',(0.,1.,0.));
#8364=DIRECTION('',(0.,0.,1.));
#8365=DIRECTION('',(0.,1.,0.));
#8366=DIRECTION('',(0.,0.,1.));
#8367=DIRECTION('center_axis',(0.,-1.,0.));
#8368=DIRECTION('ref_axis',(1.,0.,0.));
#8369=DIRECTION('',(0.,0.,1.));
#8370=DIRECTION('',(1.,0.,0.));
#8371=DIRECTION('center_axis',(0.,1.,0.));
#8372=DIRECTION('ref_axis',(-1.,0.,0.));
#8373=DIRECTION('',(-1.,0.,0.));
#8374=DIRECTION('',(0.,0.,1.));
#8375=DIRECTION('center_axis',(-1.,0.,0.));
#8376=DIRECTION('ref_axis',(0.,-1.,0.));
#8377=DIRECTION('',(0.,-1.,0.));
#8378=DIRECTION('',(0.,1.,0.));
#8379=DIRECTION('center_axis',(0.,0.,1.));
#8380=DIRECTION('ref_axis',(1.,0.,0.));
#8381=DIRECTION('center_axis',(0.,0.,1.));
#8382=DIRECTION('ref_axis',(1.,0.,0.));
#10254=CARTESIAN_POINT('',(0.,0.,0.));
#10255=CARTESIAN_POINT('Origin',(-1.06066017177982,-1.06066017177982,20.2));
#10256=CARTESIAN_POINT('',(-1.22566017177982,-1.06066017177982,20.2));
#10257=CARTESIAN_POINT('Origin',(-1.06066017177982,-1.06066017177982,20.2));
#10258=CARTESIAN_POINT('',(-1.22566017177982,-1.06066017177982,21.));
#10259=CARTESIAN_POINT('',(-1.22566017177982,-1.06066017177982,20.2));
#10260=CARTESIAN_POINT('Origin',(-1.06066017177982,-1.06066017177982,21.));
#10261=CARTESIAN_POINT('Origin',(-1.06066017177982,-1.06066017177982,20.2));
#10262=CARTESIAN_POINT('Origin',(-1.06066017177982,1.06066017177982,20.2));
#10263=CARTESIAN_POINT('',(-1.22566017177982,1.06066017177982,20.2));
#10264=CARTESIAN_POINT('Origin',(-1.06066017177982,1.06066017177982,20.2));
#10265=CARTESIAN_POINT('',(-1.22566017177982,1.06066017177982,21.));
#10266=CARTESIAN_POINT('',(-1.22566017177982,1.06066017177982,20.2));
#10267=CARTESIAN_POINT('Origin',(-1.06066017177982,1.06066017177982,21.));
#10268=CARTESIAN_POINT('Origin',(-1.06066017177982,1.06066017177982,20.2));
#10269=CARTESIAN_POINT('Origin',(1.06066017177982,1.06066017177982,20.2));
#10270=CARTESIAN_POINT('',(0.895660171779821,1.06066017177982,20.2));
#10271=CARTESIAN_POINT('Origin',(1.06066017177982,1.06066017177982,20.2));
#10272=CARTESIAN_POINT('',(0.895660171779821,1.06066017177982,21.));
#10273=CARTESIAN_POINT('',(0.895660171779821,1.06066017177982,20.2));
#10274=CARTESIAN_POINT('Origin',(1.06066017177982,1.06066017177982,21.));
#10275=CARTESIAN_POINT('Origin',(1.06066017177982,1.06066017177982,20.2));
#10276=CARTESIAN_POINT('Origin',(1.06066017177982,-1.06066017177982,20.2));
#10277=CARTESIAN_POINT('',(0.895660171779821,-1.06066017177982,20.2));
#10278=CARTESIAN_POINT('Origin',(1.06066017177982,-1.06066017177982,20.2));
#10279=CARTESIAN_POINT('',(0.895660171779821,-1.06066017177982,21.));
#10280=CARTESIAN_POINT('',(0.895660171779821,-1.06066017177982,20.2));
#10281=CARTESIAN_POINT('Origin',(1.06066017177982,-1.06066017177982,21.));
#10282=CARTESIAN_POINT('Origin',(1.06066017177982,-1.06066017177982,20.2));
#10283=CARTESIAN_POINT('Origin',(0.,0.,12.5));
#10284=CARTESIAN_POINT('',(-1.05,-1.28587913910472E-16,12.5));
#10285=CARTESIAN_POINT('Origin',(0.,0.,12.5));
#10286=CARTESIAN_POINT('',(-1.05,1.28587913910472E-16,21.));
#10287=CARTESIAN_POINT('',(-1.05,-1.28587913910472E-16,12.5));
#10288=CARTESIAN_POINT('Origin',(0.,0.,21.));
#10289=CARTESIAN_POINT('Origin',(0.,0.,12.5));
#10290=CARTESIAN_POINT('',(-0.625,-7.65404249467096E-17,12.5));
#10291=CARTESIAN_POINT('Origin',(0.,0.,12.5));
#10292=CARTESIAN_POINT('Origin',(0.,0.,10.9));
#10293=CARTESIAN_POINT('',(-0.625,-7.65404249467096E-17,11.));
#10294=CARTESIAN_POINT('Origin',(0.,0.,11.));
#10295=CARTESIAN_POINT('',(-0.625,-7.65404249467096E-17,10.9));
#10296=CARTESIAN_POINT('Origin',(3.75,0.,2.4));
#10297=CARTESIAN_POINT('',(3.25,-6.12323399573677E-17,2.4));
#10298=CARTESIAN_POINT('Origin',(3.75,0.,2.4));
#10299=CARTESIAN_POINT('',(3.25,6.12323399573677E-17,21.));
#10300=CARTESIAN_POINT('',(3.25,-6.12323399573677E-17,2.4));
#10301=CARTESIAN_POINT('Origin',(3.75,0.,21.));
#10302=CARTESIAN_POINT('Origin',(3.75,0.,2.4));
#10303=CARTESIAN_POINT('',(3.475,-3.36777869765523E-17,2.4));
#10304=CARTESIAN_POINT('Origin',(3.75,0.,2.4));
#10305=CARTESIAN_POINT('Origin',(3.75,0.,0.9));
#10306=CARTESIAN_POINT('',(3.475,-3.36777869765523E-17,1.));
#10307=CARTESIAN_POINT('Origin',(3.75,0.,1.));
#10308=CARTESIAN_POINT('',(3.475,-3.36777869765523E-17,0.9));
#10309=CARTESIAN_POINT('Origin',(-3.75,0.,2.4));
#10310=CARTESIAN_POINT('',(-4.25,-6.12323399573677E-17,2.4));
#10311=CARTESIAN_POINT('Origin',(-3.75,0.,2.4));
#10312=CARTESIAN_POINT('',(-4.25,6.12323399573677E-17,21.));
#10313=CARTESIAN_POINT('',(-4.25,-6.12323399573677E-17,2.4));
#10314=CARTESIAN_POINT('Origin',(-3.75,0.,21.));
#10315=CARTESIAN_POINT('Origin',(-3.75,0.,2.4));
#10316=CARTESIAN_POINT('',(-4.025,-3.36777869765522E-17,2.4));
#10317=CARTESIAN_POINT('Origin',(-3.75,0.,2.4));
#10318=CARTESIAN_POINT('Origin',(-3.75,0.,0.9));
#10319=CARTESIAN_POINT('',(-4.025,-3.36777869765522E-17,1.));
#10320=CARTESIAN_POINT('Origin',(-3.75,0.,1.));
#10321=CARTESIAN_POINT('',(-4.025,-3.36777869765522E-17,0.9));
#10322=CARTESIAN_POINT('Origin',(4.5,-2.,11.));
#10323=CARTESIAN_POINT('',(-4.5,1.,11.));
#10324=CARTESIAN_POINT('',(-3.,1.,11.));
#10325=CARTESIAN_POINT('',(0.75,1.,11.));
#10326=CARTESIAN_POINT('',(-4.5,2.,11.));
#10327=CARTESIAN_POINT('',(-4.5,-2.,11.));
#10328=CARTESIAN_POINT('',(4.5,2.,11.));
#10329=CARTESIAN_POINT('',(-4.5,2.,11.));
#10330=CARTESIAN_POINT('',(4.5,1.,11.));
#10331=CARTESIAN_POINT('',(4.5,-2.,11.));
#10332=CARTESIAN_POINT('',(3.,1.,11.));
#10333=CARTESIAN_POINT('',(4.125,1.,11.));
#10334=CARTESIAN_POINT('',(3.,-1.,11.));
#10335=CARTESIAN_POINT('',(3.,-1.5,11.));
#10336=CARTESIAN_POINT('',(4.5,-1.,11.));
#10337=CARTESIAN_POINT('',(4.125,-1.,11.));
#10338=CARTESIAN_POINT('',(4.5,-2.,11.));
#10339=CARTESIAN_POINT('',(4.5,-2.,11.));
#10340=CARTESIAN_POINT('',(-4.5,-2.,11.));
#10341=CARTESIAN_POINT('',(-4.5,-2.,11.));
#10342=CARTESIAN_POINT('',(-4.5,-1.,11.));
#10343=CARTESIAN_POINT('',(-4.5,-2.,11.));
#10344=CARTESIAN_POINT('',(-3.,-1.,11.));
#10345=CARTESIAN_POINT('',(0.,-1.,11.));
#10346=CARTESIAN_POINT('',(-3.,-1.5,11.));
#10347=CARTESIAN_POINT('Origin',(0.,2.,16.));
#10348=CARTESIAN_POINT('',(-4.5,2.,21.));
#10349=CARTESIAN_POINT('',(4.5,2.,21.));
#10350=CARTESIAN_POINT('',(4.5,2.,21.));
#10351=CARTESIAN_POINT('',(4.5,2.,11.));
#10352=CARTESIAN_POINT('',(-4.5,2.,21.));
#10353=CARTESIAN_POINT('Origin',(0.,-2.,16.));
#10354=CARTESIAN_POINT('',(4.5,-2.,21.));
#10355=CARTESIAN_POINT('',(-4.5,-2.,21.));
#10356=CARTESIAN_POINT('',(4.5,-2.,21.));
#10357=CARTESIAN_POINT('',(-4.5,-2.,21.));
#10358=CARTESIAN_POINT('',(4.5,-2.,11.));
#10359=CARTESIAN_POINT('Origin',(3.,-1.,1.));
#10360=CARTESIAN_POINT('',(3.,1.,1.));
#10361=CARTESIAN_POINT('',(3.,1.,21.));
#10362=CARTESIAN_POINT('',(3.,-1.,1.));
#10363=CARTESIAN_POINT('',(3.,-1.,1.));
#10364=CARTESIAN_POINT('',(3.,-1.,21.));
#10365=CARTESIAN_POINT('Origin',(3.75,1.,11.));
#10366=CARTESIAN_POINT('',(4.5,1.,1.));
#10367=CARTESIAN_POINT('',(4.5,1.,1.));
#10368=CARTESIAN_POINT('',(3.,1.,1.));
#10369=CARTESIAN_POINT('Origin',(4.5,-1.,1.));
#10370=CARTESIAN_POINT('',(4.5,-1.,1.));
#10371=CARTESIAN_POINT('',(3.,-1.,1.));
#10372=CARTESIAN_POINT('',(4.5,-1.,1.));
#10373=CARTESIAN_POINT('Origin',(4.5,-1.,21.));
#10374=CARTESIAN_POINT('',(4.5,-1.,1.));
#10375=CARTESIAN_POINT('',(4.5,-1.,21.));
#10376=CARTESIAN_POINT('Origin',(3.75,-1.,11.));
#10377=CARTESIAN_POINT('Origin',(-3.,-1.,1.));
#10378=CARTESIAN_POINT('',(-3.,-1.,1.));
#10379=CARTESIAN_POINT('',(-3.,-1.,1.));
#10380=CARTESIAN_POINT('',(-3.,1.,1.));
#10381=CARTESIAN_POINT('',(-3.,-1.,1.));
#10382=CARTESIAN_POINT('',(-3.,1.,1.));
#10383=CARTESIAN_POINT('Origin',(-4.5,-1.,1.));
#10384=CARTESIAN_POINT('',(-4.5,-1.,1.));
#10385=CARTESIAN_POINT('',(-4.5,-1.,1.));
#10386=CARTESIAN_POINT('',(-4.5,-1.,1.));
#10387=CARTESIAN_POINT('Origin',(-3.,1.,1.));
#10388=CARTESIAN_POINT('',(-4.5,1.,1.));
#10389=CARTESIAN_POINT('',(-3.,1.,1.));
#10390=CARTESIAN_POINT('',(-4.5,1.,1.));
#10391=CARTESIAN_POINT('Origin',(-4.5,1.,1.));
#10392=CARTESIAN_POINT('',(-4.5,1.,1.));
#10393=CARTESIAN_POINT('',(-4.5,-2.,21.));
#10394=CARTESIAN_POINT('Origin',(-3.75,0.,21.));
#10395=CARTESIAN_POINT('Origin',(-3.75,0.,1.));
#13201=UNCERTAINTY_MEASURE_WITH_UNIT(LENGTH_MEASURE(0.001),#13278,
'DISTANCE_ACCURACY_VALUE',
'Maximum model space distance between geometric entities at asserted c
onnectivities');
#13233=UNCERTAINTY_MEASURE_WITH_UNIT(LENGTH_MEASURE(0.001),#13278,
'DISTANCE_ACCURACY_VALUE',
'Maximum model space distance between geometric entities at asserted c
onnectivities');
#13245=(
GEOMETRIC_REPRESENTATION_CONTEXT(3)
GLOBAL_UNCERTAINTY_ASSIGNED_CONTEXT((#13201))
GLOBAL_UNIT_ASSIGNED_CONTEXT((#13278,#13280,#13281))
REPRESENTATION_CONTEXT('','3D')
);
#13277=(
GEOMETRIC_REPRESENTATION_CONTEXT(3)
GLOBAL_UNCERTAINTY_ASSIGNED_CONTEXT((#13233))
GLOBAL_UNIT_ASSIGNED_CONTEXT((#13278,#13280,#13281))
REPRESENTATION_CONTEXT('','3D')
);
#13278=(
LENGTH_UNIT()
NAMED_UNIT(*)
SI_UNIT(.CENTI.,.METRE.)
);
#13280=(
NAMED_UNIT(*)
PLANE_ANGLE_UNIT()
SI_UNIT($,.RADIAN.)
);
#13281=(
NAMED_UNIT(*)
SI_UNIT($,.STERADIAN.)
SOLID_ANGLE_UNIT()
);
#13293=SHAPE_DEFINITION_REPRESENTATION(#13336,#13450);
#13336=PRODUCT_DEFINITION_SHAPE('',$,#13494);
#13450=SHAPE_REPRESENTATION('',(#7063),#13245);
#13482=PRODUCT_DEFINITION_CONTEXT('part definition',#13613,'design');
#13494=PRODUCT_DEFINITION('Slide guide bridge','Slide guide bridge',#13537,
#13482);
#13537=PRODUCT_DEFINITION_FORMATION('',$,#13626);
#13613=APPLICATION_CONTEXT(
'Core Data for Automotive Mechanical Design Process');
#13614=PRODUCT_CONTEXT('part definition',#13613,'mechanical');
#13626=PRODUCT('Slide guide bridge','Slide guide bridge',
'Slide guide bridge',(#13614));
#13707=COLOUR_RGB('Sky Blue',0.24,0.69,0.87);
#13708=FILL_AREA_STYLE_COLOUR('',#13707);
#13709=FILL_AREA_STYLE('',(#13708));
#13710=SURFACE_STYLE_FILL_AREA(#13709);
#13711=SURFACE_SIDE_STYLE('',(#13710));
#13712=SURFACE_STYLE_USAGE(.BOTH.,#13711);
#13713=PRESENTATION_STYLE_ASSIGNMENT((#13712));
ENDSEC;
END-ISO-10303-21;
